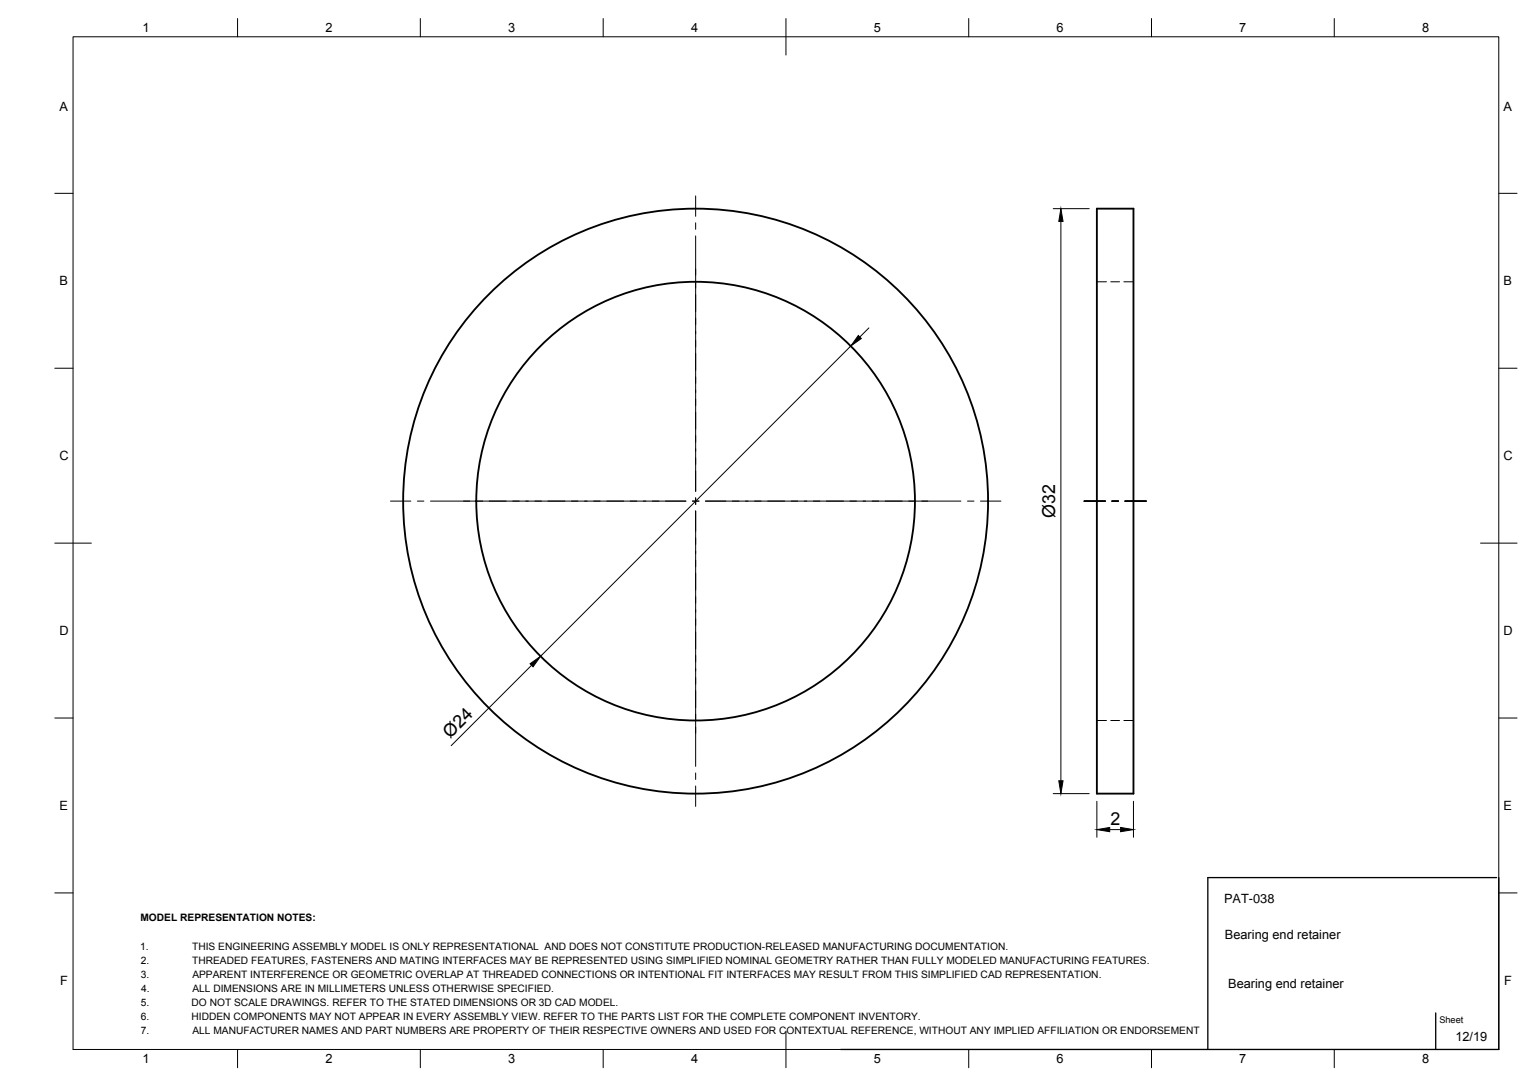
ISO-10303-21;
HEADER;
/* Generated by software containing ST-Developer
 * from STEP Tools, Inc. (www.steptools.com) 
 */

FILE_DESCRIPTION(
/* description */ ('Fork-mounted skate wheel'),
/* implementation_level */ '2;1');

FILE_NAME(
/* name */ 'Bearing end retainer.step',
/* time_stamp */ '2026-10-29T16:11:26-07:00',
/* author */ (''),
/* organization */ (''),
/* preprocessor_version */ 'ST-DEVELOPER v20.2',
/* originating_system */ 'Autodesk Translation Framework v15.17.0.0',
/* authorisation */ '');

FILE_SCHEMA (('AUTOMOTIVE_DESIGN { 1 0 10303 214 3 1 1 }'));
ENDSEC;

DATA;
#10=MECHANICAL_DESIGN_GEOMETRIC_PRESENTATION_REPRESENTATION('',(#164),#3688);
#133=SHAPE_REPRESENTATION_RELATIONSHIP('SRR','None',#3758,#145);
#145=ADVANCED_BREP_SHAPE_REPRESENTATION('',(#182),#3687);
#164=STYLED_ITEM('',(#3896),#182);
#182=MANIFOLD_SOLID_BREP('Body1',#1826);
#217=FACE_BOUND('',#535,.T.);
#218=FACE_BOUND('',#537,.T.);
#274=PLANE('',#2212);
#275=PLANE('',#2213);
#385=FACE_OUTER_BOUND('',#532,.T.);
#386=FACE_OUTER_BOUND('',#533,.T.);
#387=FACE_OUTER_BOUND('',#534,.T.);
#388=FACE_OUTER_BOUND('',#536,.T.);
#532=EDGE_LOOP('',(#1649,#1650,#1651,#1652));
#533=EDGE_LOOP('',(#1653,#1654,#1655,#1656));
#534=EDGE_LOOP('',(#1657));
#535=EDGE_LOOP('',(#1658));
#536=EDGE_LOOP('',(#1659));
#537=EDGE_LOOP('',(#1660));
#630=LINE('',#3638,#724);
#631=LINE('',#3644,#725);
#724=VECTOR('',#2809,1.2);
#725=VECTOR('',#2816,1.6);
#836=CIRCLE('',#2207,1.2);
#837=CIRCLE('',#2208,1.2);
#838=CIRCLE('',#2210,1.6);
#839=CIRCLE('',#2211,1.6);
#991=VERTEX_POINT('',#3635);
#992=VERTEX_POINT('',#3637);
#993=VERTEX_POINT('',#3641);
#994=VERTEX_POINT('',#3643);
#1211=EDGE_CURVE('',#991,#991,#836,.T.);
#1212=EDGE_CURVE('',#991,#992,#630,.T.);
#1213=EDGE_CURVE('',#992,#992,#837,.T.);
#1214=EDGE_CURVE('',#993,#993,#838,.T.);
#1215=EDGE_CURVE('',#993,#994,#631,.T.);
#1216=EDGE_CURVE('',#994,#994,#839,.T.);
#1649=ORIENTED_EDGE('',*,*,#1211,.F.);
#1650=ORIENTED_EDGE('',*,*,#1212,.T.);
#1651=ORIENTED_EDGE('',*,*,#1213,.T.);
#1652=ORIENTED_EDGE('',*,*,#1212,.F.);
#1653=ORIENTED_EDGE('',*,*,#1214,.F.);
#1654=ORIENTED_EDGE('',*,*,#1215,.T.);
#1655=ORIENTED_EDGE('',*,*,#1216,.T.);
#1656=ORIENTED_EDGE('',*,*,#1215,.F.);
#1657=ORIENTED_EDGE('',*,*,#1214,.T.);
#1658=ORIENTED_EDGE('',*,*,#1211,.T.);
#1659=ORIENTED_EDGE('',*,*,#1216,.F.);
#1660=ORIENTED_EDGE('',*,*,#1213,.F.);
#1692=CYLINDRICAL_SURFACE('',#2206,1.2);
#1693=CYLINDRICAL_SURFACE('',#2209,1.6);
#1803=ADVANCED_FACE('',(#385),#1692,.F.);
#1804=ADVANCED_FACE('',(#386),#1693,.T.);
#1805=ADVANCED_FACE('',(#387,#217),#274,.T.);
#1806=ADVANCED_FACE('',(#388,#218),#275,.F.);
#1826=CLOSED_SHELL('',(#1803,#1804,#1805,#1806));
#2205=AXIS2_PLACEMENT_3D('',#3633,#2803,#2804);
#2206=AXIS2_PLACEMENT_3D('',#3634,#2805,#2806);
#2207=AXIS2_PLACEMENT_3D('',#3636,#2807,#2808);
#2208=AXIS2_PLACEMENT_3D('',#3639,#2810,#2811);
#2209=AXIS2_PLACEMENT_3D('',#3640,#2812,#2813);
#2210=AXIS2_PLACEMENT_3D('',#3642,#2814,#2815);
#2211=AXIS2_PLACEMENT_3D('',#3645,#2817,#2818);
#2212=AXIS2_PLACEMENT_3D('',#3646,#2819,#2820);
#2213=AXIS2_PLACEMENT_3D('',#3647,#2821,#2822);
#2803=DIRECTION('axis',(0.,0.,1.));
#2804=DIRECTION('refdir',(1.,0.,0.));
#2805=DIRECTION('center_axis',(0.,1.,0.));
#2806=DIRECTION('ref_axis',(1.,0.,0.));
#2807=DIRECTION('center_axis',(0.,-1.,0.));
#2808=DIRECTION('ref_axis',(1.,0.,0.));
#2809=DIRECTION('',(0.,-1.,0.));
#2810=DIRECTION('center_axis',(0.,-1.,0.));
#2811=DIRECTION('ref_axis',(1.,0.,0.));
#2812=DIRECTION('center_axis',(0.,1.,0.));
#2813=DIRECTION('ref_axis',(1.,0.,0.));
#2814=DIRECTION('center_axis',(0.,1.,0.));
#2815=DIRECTION('ref_axis',(1.,0.,0.));
#2816=DIRECTION('',(0.,-1.,0.));
#2817=DIRECTION('center_axis',(0.,1.,0.));
#2818=DIRECTION('ref_axis',(1.,0.,0.));
#2819=DIRECTION('center_axis',(0.,1.,0.));
#2820=DIRECTION('ref_axis',(1.,0.,0.));
#2821=DIRECTION('center_axis',(0.,1.,0.));
#2822=DIRECTION('ref_axis',(1.,0.,0.));
#3633=CARTESIAN_POINT('',(0.,0.,0.));
#3634=CARTESIAN_POINT('Origin',(0.,1.1,3.5));
#3635=CARTESIAN_POINT('',(-1.2,1.3,3.5));
#3636=CARTESIAN_POINT('Origin',(0.,1.3,3.5));
#3637=CARTESIAN_POINT('',(-1.2,1.1,3.5));
#3638=CARTESIAN_POINT('',(-1.2,1.1,3.5));
#3639=CARTESIAN_POINT('Origin',(0.,1.1,3.5));
#3640=CARTESIAN_POINT('Origin',(0.,1.1,3.5));
#3641=CARTESIAN_POINT('',(-1.6,1.3,3.5));
#3642=CARTESIAN_POINT('Origin',(0.,1.3,3.5));
#3643=CARTESIAN_POINT('',(-1.6,1.1,3.5));
#3644=CARTESIAN_POINT('',(-1.6,1.1,3.5));
#3645=CARTESIAN_POINT('Origin',(0.,1.1,3.5));
#3646=CARTESIAN_POINT('Origin',(0.,1.3,3.5));
#3647=CARTESIAN_POINT('Origin',(0.,1.1,3.5));
#3670=UNCERTAINTY_MEASURE_WITH_UNIT(LENGTH_MEASURE(0.001),#3689,
'DISTANCE_ACCURACY_VALUE',
'Maximum model space distance between geometric entities at asserted c
onnectivities');
#3671=UNCERTAINTY_MEASURE_WITH_UNIT(LENGTH_MEASURE(0.001),#3689,
'DISTANCE_ACCURACY_VALUE',
'Maximum model space distance between geometric entities at asserted c
onnectivities');
#3687=(
GEOMETRIC_REPRESENTATION_CONTEXT(3)
GLOBAL_UNCERTAINTY_ASSIGNED_CONTEXT((#3670))
GLOBAL_UNIT_ASSIGNED_CONTEXT((#3689,#3691,#3692))
REPRESENTATION_CONTEXT('','3D')
);
#3688=(
GEOMETRIC_REPRESENTATION_CONTEXT(3)
GLOBAL_UNCERTAINTY_ASSIGNED_CONTEXT((#3671))
GLOBAL_UNIT_ASSIGNED_CONTEXT((#3689,#3691,#3692))
REPRESENTATION_CONTEXT('','3D')
);
#3689=(
LENGTH_UNIT()
NAMED_UNIT(*)
SI_UNIT(.CENTI.,.METRE.)
);
#3691=(
NAMED_UNIT(*)
PLANE_ANGLE_UNIT()
SI_UNIT($,.RADIAN.)
);
#3692=(
NAMED_UNIT(*)
SI_UNIT($,.STERADIAN.)
SOLID_ANGLE_UNIT()
);
#3708=SHAPE_DEFINITION_REPRESENTATION(#3735,#3758);
#3735=PRODUCT_DEFINITION_SHAPE('',$,#3775);
#3758=SHAPE_REPRESENTATION('',(#2205),#3687);
#3759=PRODUCT_DEFINITION_CONTEXT('part definition',#3809,'design');
#3775=PRODUCT_DEFINITION('Bearing end retainer','Bearing end retainer',
#3791,#3759);
#3791=PRODUCT_DEFINITION_FORMATION('',$,#3826);
#3809=APPLICATION_CONTEXT(
'Core Data for Automotive Mechanical Design Process');
#3810=PRODUCT_CONTEXT('part definition',#3809,'mechanical');
#3826=PRODUCT('Bearing end retainer','Bearing end retainer',
'Bearing end retainer',(#3810));
#3890=COLOUR_RGB('Grey',0.48,0.52,0.57);
#3891=FILL_AREA_STYLE_COLOUR('',#3890);
#3892=FILL_AREA_STYLE('',(#3891));
#3893=SURFACE_STYLE_FILL_AREA(#3892);
#3894=SURFACE_SIDE_STYLE('',(#3893));
#3895=SURFACE_STYLE_USAGE(.BOTH.,#3894);
#3896=PRESENTATION_STYLE_ASSIGNMENT((#3895));
ENDSEC;
END-ISO-10303-21;
